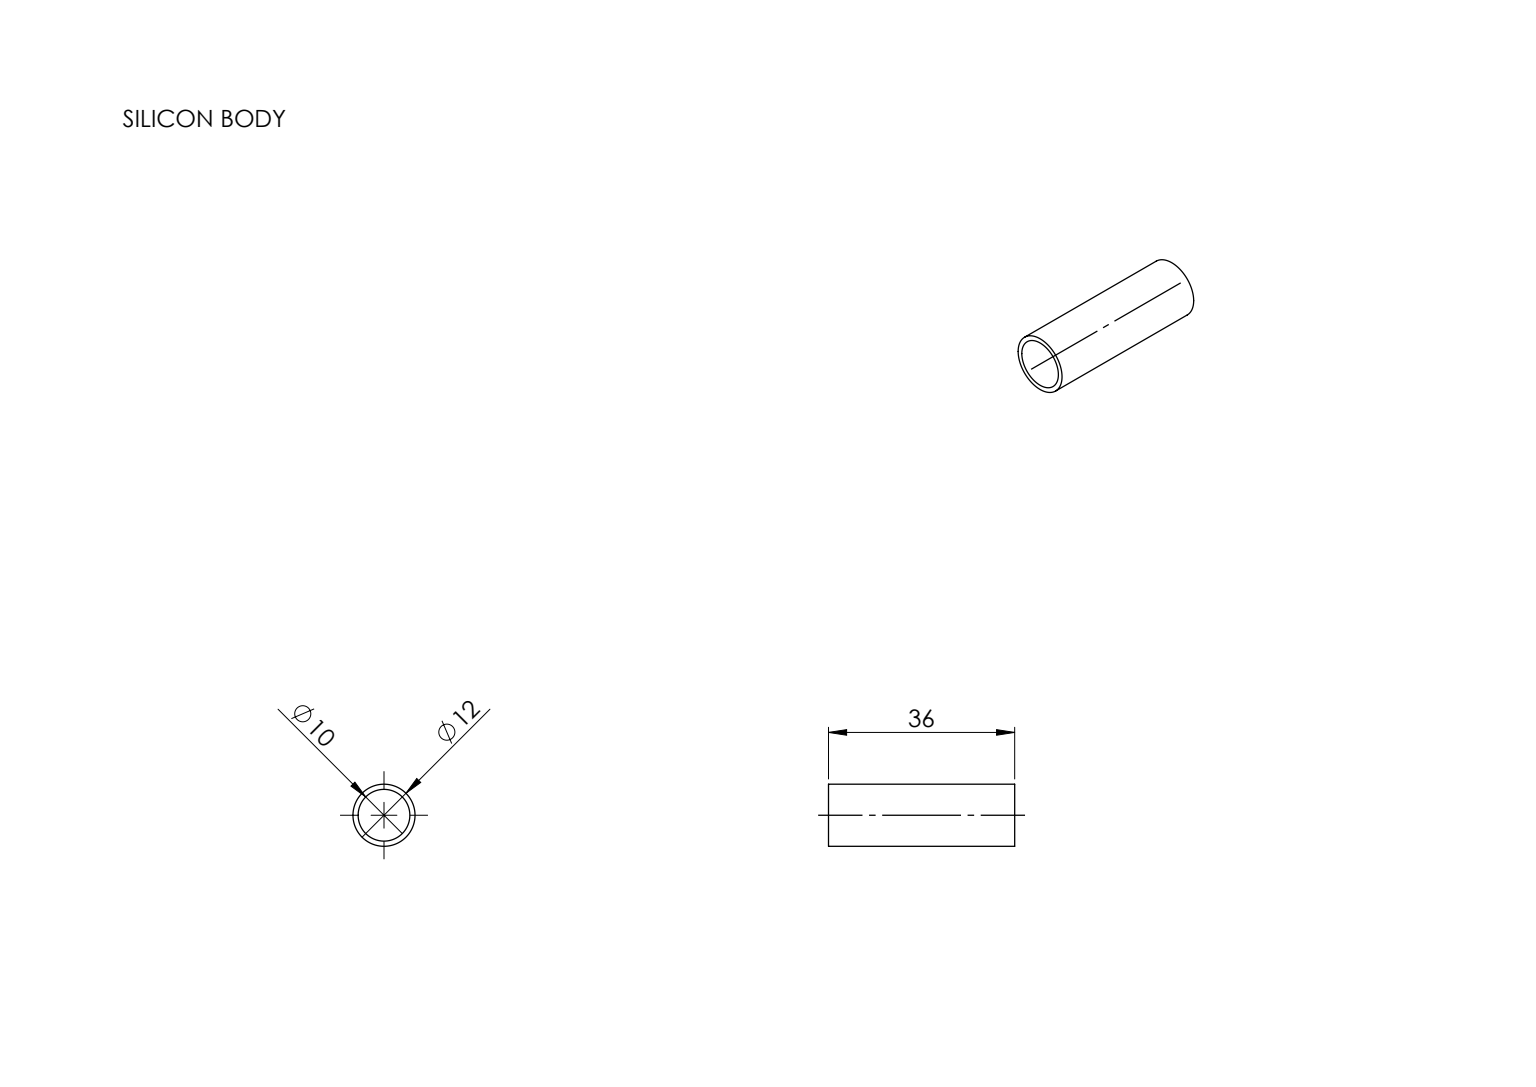
ISO-10303-21;
HEADER;
FILE_DESCRIPTION (('STEP AP214'),
    '1' );
FILE_NAME ('silicon body.step',
    '2026-10-04T10:31:01',
    ( '' ),
    ( '' ),
    'SwSTEP 2.0',
    'SolidWorks 2026',
    '' );
FILE_SCHEMA (( 'AUTOMOTIVE_DESIGN' ));
ENDSEC;

DATA;
#110=UNCERTAINTY_MEASURE_WITH_UNIT (LENGTH_MEASURE( 1.000000000000000082E-05 ), #6665, 'distance_accuracy_value', 'NONE');
#144=ORIENTED_EDGE ( 'NONE', *, *, #8868, .F. ) ;
#242=PLANE ( 'NONE',  #13414 ) ;
#448=CARTESIAN_POINT ( 'NONE',  ( 5.000000000000000000, 6.123233995736765296E-16, 52.97056274847714263 ) ) ;
#638=CARTESIAN_POINT ( 'NONE',  ( 6.000000000000000000, 7.347880794884118750E-16, 36.00000000000000711 ) ) ;
#660=VERTEX_POINT ( 'NONE', #9125 ) ;
#661=CARTESIAN_POINT ( 'NONE',  ( 5.000000000000000000, 6.123233995736765296E-16, 0.000000000000000000 ) ) ;
#724=( GEOMETRIC_REPRESENTATION_CONTEXT ( 3 ) GLOBAL_UNCERTAINTY_ASSIGNED_CONTEXT ( ( #15717 ) ) GLOBAL_UNIT_ASSIGNED_CONTEXT ( ( #11873, #5266, #3102 ) ) REPRESENTATION_CONTEXT ( 'NONE', 'WORKASPACE' ) );
#773=DIRECTION ( 'NONE',  ( -1.000000000000000000, 0.000000000000000000, 0.000000000000000000 ) ) ;
#850=FACE_OUTER_BOUND ( 'NONE', #8632, .T. ) ;
#1160=DIRECTION ( 'NONE',  ( 0.000000000000000000, 0.000000000000000000, -1.000000000000000000 ) ) ;
#1215=ORIENTED_EDGE ( 'NONE', *, *, #13936, .T. ) ;
#1216=EDGE_CURVE ( 'NONE', #4645, #660, #6788, .T. ) ;
#1314=CIRCLE ( 'NONE', #7917, 6.000000000000000000 ) ;
#1315=CARTESIAN_POINT ( 'NONE',  ( -5.000000000000000000, 0.000000000000000000, 52.97056274847714263 ) ) ;
#1324=EDGE_CURVE ( 'NONE', #3143, #14086, #11349, .T. ) ;
#1369=EDGE_LOOP ( 'NONE', ( #1607, #4828, #4050, #11315 ) ) ;
#1521=PLANE ( 'NONE',  #8777 ) ;
#1558=( NAMED_UNIT ( * ) SI_UNIT ( $, .STERADIAN. ) SOLID_ANGLE_UNIT ( ) );
#1607=ORIENTED_EDGE ( 'NONE', *, *, #15050, .F. ) ;
#1651=DIRECTION ( 'NONE',  ( 1.000000000000000000, 0.000000000000000000, 0.000000000000000000 ) ) ;
#1793=PRODUCT_DEFINITION_CONTEXT ( 'detailed design', #15421, 'design' ) ;
#2339=FACE_OUTER_BOUND ( 'NONE', #9666, .T. ) ;
#2377=FACE_OUTER_BOUND ( 'NONE', #14707, .T. ) ;
#2413=CLOSED_SHELL ( 'NONE', ( #10324, #3176, #13081, #10084, #10515, #11545 ) ) ;
#2510=MECHANICAL_DESIGN_GEOMETRIC_PRESENTATION_REPRESENTATION('',(#7844),#724);
#2605=ORIENTED_EDGE ( 'NONE', *, *, #14901, .F. ) ;
#2623=CARTESIAN_POINT ( 'NONE',  ( 0.000000000000000000, 0.000000000000000000, 36.00000000000000711 ) ) ;
#2712=FILL_AREA_STYLE ('',( #3685 ) ) ;
#2884=ORIENTED_EDGE ( 'NONE', *, *, #6115, .T. ) ;
#2888=ORIENTED_EDGE ( 'NONE', *, *, #11475, .T. ) ;
#2907=CIRCLE ( 'NONE', #4951, 5.000000000000000000 ) ;
#2946=DIRECTION ( 'NONE',  ( 1.000000000000000000, 0.000000000000000000, 0.000000000000000000 ) ) ;
#2963=AXIS2_PLACEMENT_3D ( 'NONE', #12714, #3017, #3324 ) ;
#2994=( GEOMETRIC_REPRESENTATION_CONTEXT ( 3 ) GLOBAL_UNCERTAINTY_ASSIGNED_CONTEXT ( ( #6009 ) ) GLOBAL_UNIT_ASSIGNED_CONTEXT ( ( #6118, #10880, #9860 ) ) REPRESENTATION_CONTEXT ( 'NONE', 'WORKASPACE' ) );
#3015=AXIS2_PLACEMENT_3D ( 'NONE', #13723, #13797, #8655 ) ;
#3017=DIRECTION ( 'NONE',  ( 0.000000000000000000, 0.000000000000000000, 1.000000000000000000 ) ) ;
#3059=SHAPE_REPRESENTATION ( 'silicon body', ( #14201 ), #2994 ) ;
#3102=( NAMED_UNIT ( * ) SI_UNIT ( $, .STERADIAN. ) SOLID_ANGLE_UNIT ( ) );
#3142=DIRECTION ( 'NONE',  ( 1.000000000000000000, 0.000000000000000000, 0.000000000000000000 ) ) ;
#3143=VERTEX_POINT ( 'NONE', #14281 ) ;
#3176=ADVANCED_FACE ( 'NONE', ( #850 ), #7066, .T. ) ;
#3208=VERTEX_POINT ( 'NONE', #10486 ) ;
#3234=PRODUCT_DEFINITION_FORMATION_WITH_SPECIFIED_SOURCE ( 'ANY', '', #6900, .NOT_KNOWN. ) ;
#3324=DIRECTION ( 'NONE',  ( 1.000000000000000000, 0.000000000000000000, 0.000000000000000000 ) ) ;
#3577=DIRECTION ( 'NONE',  ( -1.000000000000000000, 0.000000000000000000, 0.000000000000000000 ) ) ;
#3685=FILL_AREA_STYLE_COLOUR ( '', #14474 ) ;
#3762=AXIS2_PLACEMENT_3D ( 'NONE', #15415, #13017, #773 ) ;
#3820=ORIENTED_EDGE ( 'NONE', *, *, #1216, .F. ) ;
#3931=APPLICATION_CONTEXT ( 'automotive_design' ) ;
#4009=CIRCLE ( 'NONE', #8337, 6.000000000000000000 ) ;
#4022=FILL_AREA_STYLE ('',( #5074 ) ) ;
#4050=ORIENTED_EDGE ( 'NONE', *, *, #14901, .T. ) ;
#4296=VECTOR ( 'NONE', #8334, 1000.000000000000000 ) ;
#4375=LINE ( 'NONE', #9446, #12676 ) ;
#4424=DIRECTION ( 'NONE',  ( -1.000000000000000000, 0.000000000000000000, 0.000000000000000000 ) ) ;
#4572=SURFACE_STYLE_USAGE ( .BOTH. , #15474 ) ;
#4645=VERTEX_POINT ( 'NONE', #15158 ) ;
#4739=CYLINDRICAL_SURFACE ( 'NONE', #10811, 5.000000000000000000 ) ;
#4828=ORIENTED_EDGE ( 'NONE', *, *, #8868, .T. ) ;
#4889=MANIFOLD_SOLID_BREP ( 'Extrude-Thin1', #2413 ) ;
#4951=AXIS2_PLACEMENT_3D ( 'NONE', #10470, #15324, #4424 ) ;
#4970=ORIENTED_EDGE ( 'NONE', *, *, #13089, .F. ) ;
#5074=FILL_AREA_STYLE_COLOUR ( '', #9398 ) ;
#5078=DIRECTION ( 'NONE',  ( 0.000000000000000000, 0.000000000000000000, -1.000000000000000000 ) ) ;
#5104=DIRECTION ( 'NONE',  ( 0.000000000000000000, 0.000000000000000000, 1.000000000000000000 ) ) ;
#5122=VECTOR ( 'NONE', #1160, 1000.000000000000000 ) ;
#5151=SURFACE_SIDE_STYLE ('',( #12613 ) ) ;
#5266=( NAMED_UNIT ( * ) PLANE_ANGLE_UNIT ( ) SI_UNIT ( $, .RADIAN. ) );
#5343=DIRECTION ( 'NONE',  ( -1.000000000000000000, 0.000000000000000000, 0.000000000000000000 ) ) ;
#5348=VERTEX_POINT ( 'NONE', #7701 ) ;
#5366=ORIENTED_EDGE ( 'NONE', *, *, #13936, .F. ) ;
#5612=EDGE_CURVE ( 'NONE', #3208, #5348, #6113, .T. ) ;
#5688=AXIS2_PLACEMENT_3D ( 'NONE', #8361, #8442, #6053 ) ;
#5825=AXIS2_PLACEMENT_3D ( 'NONE', #7839, #6966, #3142 ) ;
#5867=DIRECTION ( 'NONE',  ( 0.000000000000000000, 0.000000000000000000, -1.000000000000000000 ) ) ;
#5976=DIRECTION ( 'NONE',  ( 0.000000000000000000, 0.000000000000000000, -1.000000000000000000 ) ) ;
#6009=UNCERTAINTY_MEASURE_WITH_UNIT (LENGTH_MEASURE( 1.000000000000000082E-05 ), #6118, 'distance_accuracy_value', 'NONE');
#6053=DIRECTION ( 'NONE',  ( -1.000000000000000000, 0.000000000000000000, 0.000000000000000000 ) ) ;
#6113=LINE ( 'NONE', #1315, #5122 ) ;
#6115=EDGE_CURVE ( 'NONE', #660, #4645, #1314, .T. ) ;
#6118=( LENGTH_UNIT ( ) NAMED_UNIT ( * ) SI_UNIT ( .MILLI., .METRE. ) );
#6316=FACE_OUTER_BOUND ( 'NONE', #11467, .T. ) ;
#6383=FACE_OUTER_BOUND ( 'NONE', #14422, .T. ) ;
#6397=DIRECTION ( 'NONE',  ( 0.000000000000000000, 0.000000000000000000, -1.000000000000000000 ) ) ;
#6573=AXIS2_PLACEMENT_3D ( 'NONE', #8767, #13676, #7794 ) ;
#6665=( LENGTH_UNIT ( ) NAMED_UNIT ( * ) SI_UNIT ( .MILLI., .METRE. ) );
#6680=CARTESIAN_POINT ( 'NONE',  ( 0.000000000000000000, 0.000000000000000000, 0.000000000000000000 ) ) ;
#6723=SHAPE_DEFINITION_REPRESENTATION ( #9705, #3059 ) ;
#6742=SURFACE_STYLE_USAGE ( .BOTH. , #5151 ) ;
#6788=CIRCLE ( 'NONE', #2963, 6.000000000000000000 ) ;
#6880=PRODUCT_CONTEXT ( 'NONE', #3931, 'mechanical' ) ;
#6900=PRODUCT ( 'silicon body', 'silicon body', '', ( #6880 ) ) ;
#6966=DIRECTION ( 'NONE',  ( 0.000000000000000000, 0.000000000000000000, 1.000000000000000000 ) ) ;
#7063=CARTESIAN_POINT ( 'NONE',  ( 0.000000000000000000, 0.000000000000000000, 0.000000000000000000 ) ) ;
#7066=CYLINDRICAL_SURFACE ( 'NONE', #3762, 6.000000000000000000 ) ;
#7564=SURFACE_STYLE_FILL_AREA ( #2712 ) ;
#7610=SHAPE_REPRESENTATION_RELATIONSHIP ( 'NONE' , 'NONE' ,  #3059, #10306 ) ;
#7701=CARTESIAN_POINT ( 'NONE',  ( -5.000000000000000000, 0.000000000000000000, 0.000000000000000000 ) ) ;
#7715=FACE_BOUND ( 'NONE', #12704, .T. ) ;
#7794=DIRECTION ( 'NONE',  ( 1.000000000000000000, 0.000000000000000000, 0.000000000000000000 ) ) ;
#7839=CARTESIAN_POINT ( 'NONE',  ( 0.000000000000000000, 0.000000000000000000, 0.000000000000000000 ) ) ;
#7842=CIRCLE ( 'NONE', #3015, 5.000000000000000000 ) ;
#7844=STYLED_ITEM ( 'NONE', ( #9423 ), #4889 ) ;
#7878=CARTESIAN_POINT ( 'NONE',  ( 0.000000000000000000, 0.000000000000000000, 36.00000000000000711 ) ) ;
#7917=AXIS2_PLACEMENT_3D ( 'NONE', #7063, #13995, #7957 ) ;
#7957=DIRECTION ( 'NONE',  ( 1.000000000000000000, 0.000000000000000000, 0.000000000000000000 ) ) ;
#8085=CIRCLE ( 'NONE', #6573, 5.000000000000000000 ) ;
#8334=DIRECTION ( 'NONE',  ( 0.000000000000000000, 0.000000000000000000, -1.000000000000000000 ) ) ;
#8337=AXIS2_PLACEMENT_3D ( 'NONE', #7878, #12719, #5343 ) ;
#8361=CARTESIAN_POINT ( 'NONE',  ( 0.000000000000000000, 0.000000000000000000, 52.97056274847714263 ) ) ;
#8442=DIRECTION ( 'NONE',  ( 0.000000000000000000, 0.000000000000000000, -1.000000000000000000 ) ) ;
#8477=ORIENTED_EDGE ( 'NONE', *, *, #12999, .F. ) ;
#8582=CARTESIAN_POINT ( 'NONE',  ( 6.000000000000000000, 7.347880794884118750E-16, 52.97056274847714263 ) ) ;
#8632=EDGE_LOOP ( 'NONE', ( #11123, #10421, #2884, #2605 ) ) ;
#8653=( GEOMETRIC_REPRESENTATION_CONTEXT ( 3 ) GLOBAL_UNCERTAINTY_ASSIGNED_CONTEXT ( ( #110 ) ) GLOBAL_UNIT_ASSIGNED_CONTEXT ( ( #6665, #11575, #1558 ) ) REPRESENTATION_CONTEXT ( 'NONE', 'WORKASPACE' ) );
#8655=DIRECTION ( 'NONE',  ( -1.000000000000000000, 0.000000000000000000, 0.000000000000000000 ) ) ;
#8767=CARTESIAN_POINT ( 'NONE',  ( 0.000000000000000000, 0.000000000000000000, 0.000000000000000000 ) ) ;
#8777=AXIS2_PLACEMENT_3D ( 'NONE', #13536, #6397, #11153 ) ;
#8868=EDGE_CURVE ( 'NONE', #9099, #9480, #13290, .T. ) ;
#9099=VERTEX_POINT ( 'NONE', #638 ) ;
#9109=DIRECTION ( 'NONE',  ( 0.000000000000000000, 0.000000000000000000, -1.000000000000000000 ) ) ;
#9125=CARTESIAN_POINT ( 'NONE',  ( 6.000000000000000000, 7.347880794884118750E-16, 0.000000000000000000 ) ) ;
#9350=DIRECTION ( 'NONE',  ( -1.000000000000000000, 0.000000000000000000, 0.000000000000000000 ) ) ;
#9398=COLOUR_RGB ( '', 0.09019608, 0.27058824, 0.51372549) ;
#9423=PRESENTATION_STYLE_ASSIGNMENT (( #4572 ) ) ;
#9446=CARTESIAN_POINT ( 'NONE',  ( -6.000000000000000000, 0.000000000000000000, 52.97056274847714263 ) ) ;
#9480=VERTEX_POINT ( 'NONE', #14959 ) ;
#9574=VECTOR ( 'NONE', #5078, 1000.000000000000000 ) ;
#9666=EDGE_LOOP ( 'NONE', ( #9727, #5366, #15237, #13699 ) ) ;
#9705=PRODUCT_DEFINITION_SHAPE ( 'NONE', 'NONE',  #14597 ) ;
#9727=ORIENTED_EDGE ( 'NONE', *, *, #1324, .F. ) ;
#9860=( NAMED_UNIT ( * ) SI_UNIT ( $, .STERADIAN. ) SOLID_ANGLE_UNIT ( ) );
#9862=ORIENTED_EDGE ( 'NONE', *, *, #5612, .F. ) ;
#10084=ADVANCED_FACE ( 'NONE', ( #13785 ), #10292, .T. ) ;
#10215=CARTESIAN_POINT ( 'NONE',  ( 0.000000000000000000, 0.000000000000000000, 52.97056274847714263 ) ) ;
#10292=CYLINDRICAL_SURFACE ( 'NONE', #11267, 6.000000000000000000 ) ;
#10306=ADVANCED_BREP_SHAPE_REPRESENTATION ( '', ( #4889, #14201 ), #2994 ) ;
#10324=ADVANCED_FACE ( 'NONE', ( #2377 ), #15675, .F. ) ;
#10421=ORIENTED_EDGE ( 'NONE', *, *, #15050, .T. ) ;
#10470=CARTESIAN_POINT ( 'NONE',  ( 0.000000000000000000, 0.000000000000000000, 36.00000000000000711 ) ) ;
#10486=CARTESIAN_POINT ( 'NONE',  ( -5.000000000000000000, 0.000000000000000000, 36.00000000000000711 ) ) ;
#10515=ADVANCED_FACE ( 'NONE', ( #2339 ), #4739, .F. ) ;
#10811=AXIS2_PLACEMENT_3D ( 'NONE', #13318, #15637, #9350 ) ;
#10880=( NAMED_UNIT ( * ) PLANE_ANGLE_UNIT ( ) SI_UNIT ( $, .RADIAN. ) );
#11074=FACE_BOUND ( 'NONE', #14943, .T. ) ;
#11123=ORIENTED_EDGE ( 'NONE', *, *, #12999, .T. ) ;
#11153=DIRECTION ( 'NONE',  ( -1.000000000000000000, 0.000000000000000000, 0.000000000000000000 ) ) ;
#11256=AXIS2_PLACEMENT_3D ( 'NONE', #2623, #5976, #3577 ) ;
#11267=AXIS2_PLACEMENT_3D ( 'NONE', #10215, #9109, #13938 ) ;
#11315=ORIENTED_EDGE ( 'NONE', *, *, #1216, .T. ) ;
#11349=LINE ( 'NONE', #448, #9574 ) ;
#11465=ORIENTED_EDGE ( 'NONE', *, *, #13089, .T. ) ;
#11467=EDGE_LOOP ( 'NONE', ( #8477, #144 ) ) ;
#11475=EDGE_CURVE ( 'NONE', #3143, #3208, #2907, .T. ) ;
#11513=DIRECTION ( 'NONE',  ( 0.000000000000000000, 0.000000000000000000, 1.000000000000000000 ) ) ;
#11545=ADVANCED_FACE ( 'NONE', ( #11074, #6316 ), #1521, .F. ) ;
#11575=( NAMED_UNIT ( * ) PLANE_ANGLE_UNIT ( ) SI_UNIT ( $, .RADIAN. ) );
#11674=MECHANICAL_DESIGN_GEOMETRIC_PRESENTATION_REPRESENTATION('',(#12941),#8653);
#11873=( LENGTH_UNIT ( ) NAMED_UNIT ( * ) SI_UNIT ( .MILLI., .METRE. ) );
#12613=SURFACE_STYLE_FILL_AREA ( #4022 ) ;
#12676=VECTOR ( 'NONE', #5867, 1000.000000000000000 ) ;
#12704=EDGE_LOOP ( 'NONE', ( #11465, #15134 ) ) ;
#12714=CARTESIAN_POINT ( 'NONE',  ( 0.000000000000000000, 0.000000000000000000, 0.000000000000000000 ) ) ;
#12719=DIRECTION ( 'NONE',  ( 0.000000000000000000, 0.000000000000000000, -1.000000000000000000 ) ) ;
#12735=ORIENTED_EDGE ( 'NONE', *, *, #6115, .F. ) ;
#12941=STYLED_ITEM ( 'NONE', ( #15015 ), #10306 ) ;
#12999=EDGE_CURVE ( 'NONE', #9480, #9099, #4009, .T. ) ;
#13017=DIRECTION ( 'NONE',  ( 0.000000000000000000, 0.000000000000000000, -1.000000000000000000 ) ) ;
#13081=ADVANCED_FACE ( 'NONE', ( #6383, #7715 ), #242, .F. ) ;
#13089=EDGE_CURVE ( 'NONE', #5348, #14086, #8085, .T. ) ;
#13217=ORIENTED_EDGE ( 'NONE', *, *, #1324, .T. ) ;
#13290=CIRCLE ( 'NONE', #11256, 6.000000000000000000 ) ;
#13318=CARTESIAN_POINT ( 'NONE',  ( 0.000000000000000000, 0.000000000000000000, 52.97056274847714263 ) ) ;
#13414=AXIS2_PLACEMENT_3D ( 'NONE', #13834, #5104, #2946 ) ;
#13536=CARTESIAN_POINT ( 'NONE',  ( 0.000000000000000000, 0.000000000000000000, 36.00000000000000711 ) ) ;
#13676=DIRECTION ( 'NONE',  ( 0.000000000000000000, 0.000000000000000000, 1.000000000000000000 ) ) ;
#13699=ORIENTED_EDGE ( 'NONE', *, *, #15250, .F. ) ;
#13723=CARTESIAN_POINT ( 'NONE',  ( 0.000000000000000000, 0.000000000000000000, 36.00000000000000711 ) ) ;
#13785=FACE_OUTER_BOUND ( 'NONE', #1369, .T. ) ;
#13797=DIRECTION ( 'NONE',  ( 0.000000000000000000, 0.000000000000000000, -1.000000000000000000 ) ) ;
#13834=CARTESIAN_POINT ( 'NONE',  ( 0.000000000000000000, 0.000000000000000000, 0.000000000000000000 ) ) ;
#13936=EDGE_CURVE ( 'NONE', #3208, #3143, #7842, .T. ) ;
#13938=DIRECTION ( 'NONE',  ( -1.000000000000000000, 0.000000000000000000, 0.000000000000000000 ) ) ;
#13995=DIRECTION ( 'NONE',  ( 0.000000000000000000, 0.000000000000000000, 1.000000000000000000 ) ) ;
#14086=VERTEX_POINT ( 'NONE', #661 ) ;
#14201=AXIS2_PLACEMENT_3D ( 'NONE', #6680, #11513, #1651 ) ;
#14281=CARTESIAN_POINT ( 'NONE',  ( 5.000000000000000000, 6.123233995736765296E-16, 36.00000000000000711 ) ) ;
#14422=EDGE_LOOP ( 'NONE', ( #3820, #12735 ) ) ;
#14474=COLOUR_RGB ( '', 0.09019608, 0.27058824, 0.51372549) ;
#14597=PRODUCT_DEFINITION ( 'UNKNOWN', '', #3234, #1793 ) ;
#14652=ORIENTED_EDGE ( 'NONE', *, *, #11475, .F. ) ;
#14707=EDGE_LOOP ( 'NONE', ( #14652, #13217, #4970, #9862 ) ) ;
#14901=EDGE_CURVE ( 'NONE', #9480, #4645, #4375, .T. ) ;
#14943=EDGE_LOOP ( 'NONE', ( #1215, #2888 ) ) ;
#14959=CARTESIAN_POINT ( 'NONE',  ( -6.000000000000000000, 0.000000000000000000, 36.00000000000000711 ) ) ;
#15015=PRESENTATION_STYLE_ASSIGNMENT (( #6742 ) ) ;
#15050=EDGE_CURVE ( 'NONE', #9099, #660, #15574, .T. ) ;
#15134=ORIENTED_EDGE ( 'NONE', *, *, #15250, .T. ) ;
#15158=CARTESIAN_POINT ( 'NONE',  ( -6.000000000000000000, 0.000000000000000000, 0.000000000000000000 ) ) ;
#15237=ORIENTED_EDGE ( 'NONE', *, *, #5612, .T. ) ;
#15250=EDGE_CURVE ( 'NONE', #14086, #5348, #15481, .T. ) ;
#15324=DIRECTION ( 'NONE',  ( 0.000000000000000000, 0.000000000000000000, -1.000000000000000000 ) ) ;
#15415=CARTESIAN_POINT ( 'NONE',  ( 0.000000000000000000, 0.000000000000000000, 52.97056274847714263 ) ) ;
#15421=APPLICATION_CONTEXT ( 'automotive_design' ) ;
#15474=SURFACE_SIDE_STYLE ('',( #7564 ) ) ;
#15481=CIRCLE ( 'NONE', #5825, 5.000000000000000000 ) ;
#15574=LINE ( 'NONE', #8582, #4296 ) ;
#15637=DIRECTION ( 'NONE',  ( 0.000000000000000000, 0.000000000000000000, -1.000000000000000000 ) ) ;
#15675=CYLINDRICAL_SURFACE ( 'NONE', #5688, 5.000000000000000000 ) ;
#15717=UNCERTAINTY_MEASURE_WITH_UNIT (LENGTH_MEASURE( 1.000000000000000082E-05 ), #11873, 'distance_accuracy_value', 'NONE');
ENDSEC;
END-ISO-10303-21;
